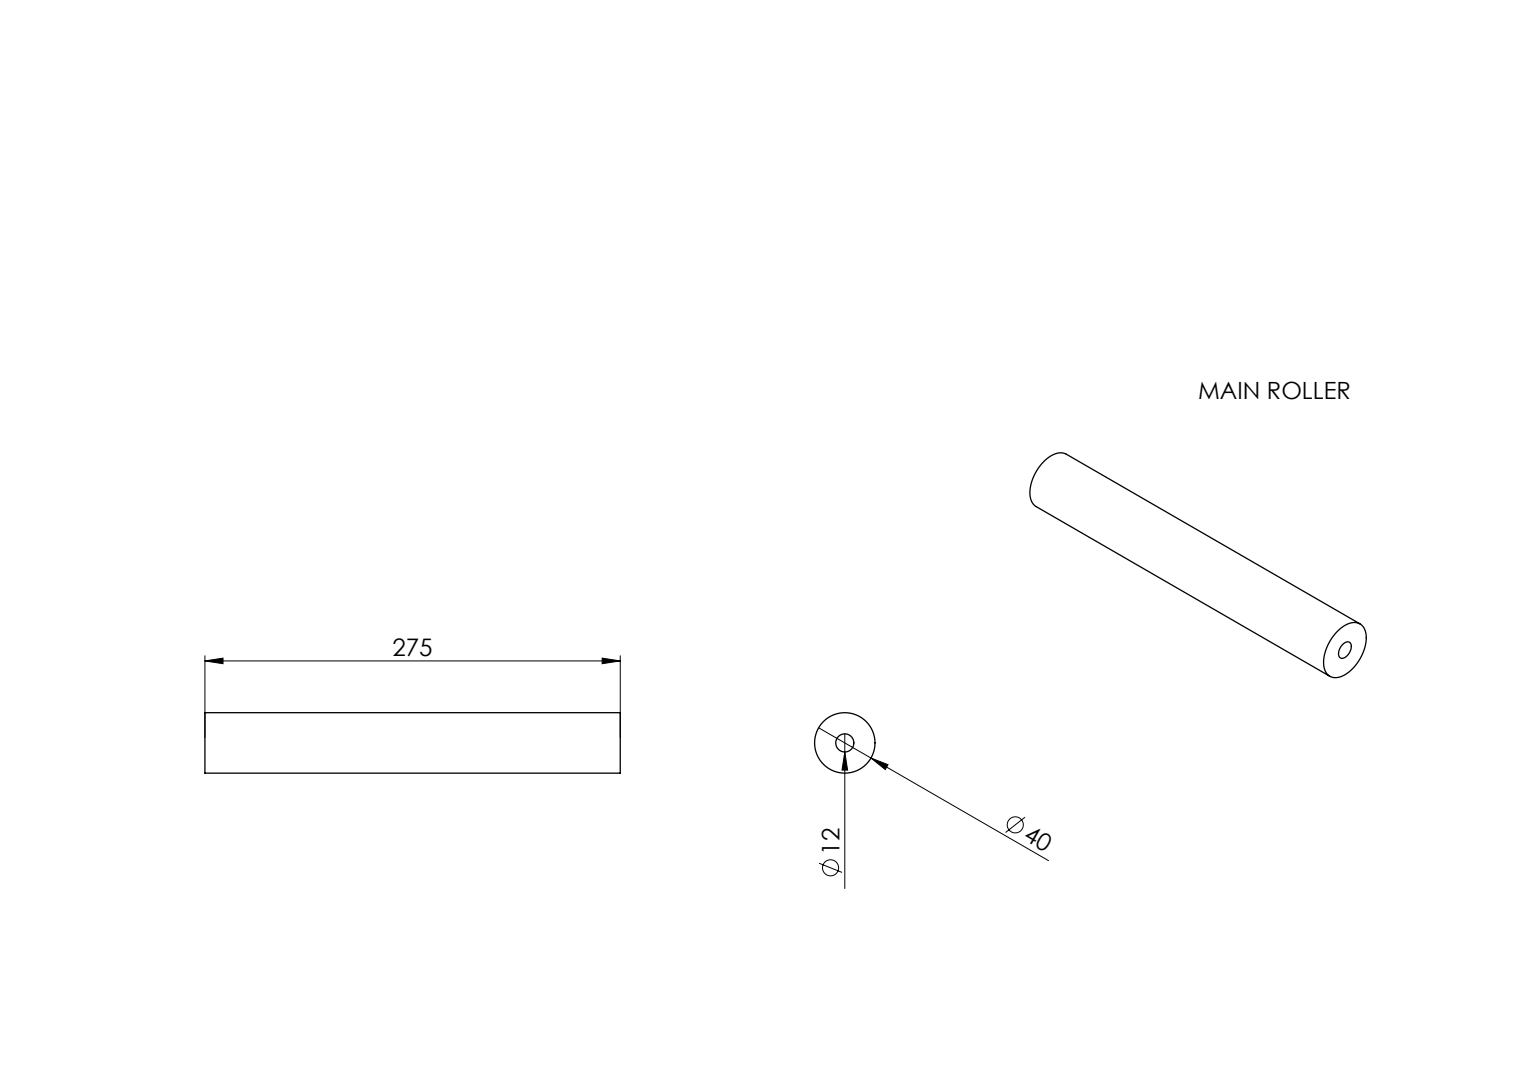
ISO-10303-21;
HEADER;
FILE_DESCRIPTION (('STEP AP214'),
    '1' );
FILE_NAME ('main roller.step',
    '2026-10-22T16:49:52',
    ( '' ),
    ( '' ),
    'SwSTEP 2.0',
    'SolidWorks 2026',
    '' );
FILE_SCHEMA (( 'AUTOMOTIVE_DESIGN' ));
ENDSEC;

DATA;
#49=CIRCLE ( 'NONE', #3968, 20.00000000000001421 ) ;
#63=CARTESIAN_POINT ( 'NONE',  ( 137.5000000000000000, 870.0000000000000000, 6.000000000000006217 ) ) ;
#76=CIRCLE ( 'NONE', #4758, 20.00000000000001421 ) ;
#77=AXIS2_PLACEMENT_3D ( 'NONE', #4332, #3953, #3470 ) ;
#109=APPLICATION_CONTEXT ( 'automotive_design' ) ;
#143=DIRECTION ( 'NONE',  ( 0.000000000000000000, 0.000000000000000000, -1.000000000000000000 ) ) ;
#179=EDGE_CURVE ( 'NONE', #353, #1195, #2907, .T. ) ;
#227=( GEOMETRIC_REPRESENTATION_CONTEXT ( 3 ) GLOBAL_UNCERTAINTY_ASSIGNED_CONTEXT ( ( #1775 ) ) GLOBAL_UNIT_ASSIGNED_CONTEXT ( ( #3570, #5196, #2363 ) ) REPRESENTATION_CONTEXT ( 'NONE', 'WORKASPACE' ) );
#245=CIRCLE ( 'NONE', #77, 6.000000000000006217 ) ;
#255=PRODUCT_DEFINITION ( 'UNKNOWN', '', #483, #2329 ) ;
#273=VERTEX_POINT ( 'NONE', #4446 ) ;
#291=EDGE_LOOP ( 'NONE', ( #3664, #547 ) ) ;
#309=CARTESIAN_POINT ( 'NONE',  ( -137.5000000000000000, 870.0000000000000000, 0.000000000000000000 ) ) ;
#332=DIRECTION ( 'NONE',  ( 0.000000000000000000, 0.000000000000000000, -1.000000000000000000 ) ) ;
#353=VERTEX_POINT ( 'NONE', #1576 ) ;
#387=ADVANCED_BREP_SHAPE_REPRESENTATION ( '', ( #3628, #4154 ), #755 ) ;
#405=MECHANICAL_DESIGN_GEOMETRIC_PRESENTATION_REPRESENTATION('',(#1277),#227);
#417=ORIENTED_EDGE ( 'NONE', *, *, #3310, .F. ) ;
#435=EDGE_CURVE ( 'NONE', #3050, #273, #1180, .T. ) ;
#479=ORIENTED_EDGE ( 'NONE', *, *, #5292, .T. ) ;
#483=PRODUCT_DEFINITION_FORMATION_WITH_SPECIFIED_SOURCE ( 'ANY', '', #4971, .NOT_KNOWN. ) ;
#496=FACE_BOUND ( 'NONE', #2841, .T. ) ;
#538=DIRECTION ( 'NONE',  ( 1.000000000000000000, 0.000000000000000000, 0.000000000000000000 ) ) ;
#547=ORIENTED_EDGE ( 'NONE', *, *, #2794, .F. ) ;
#562=VECTOR ( 'NONE', #3463, 1000.000000000000000 ) ;
#580=CARTESIAN_POINT ( 'NONE',  ( 137.5000000000000000, 870.0000000000000000, 0.000000000000000000 ) ) ;
#755=( GEOMETRIC_REPRESENTATION_CONTEXT ( 3 ) GLOBAL_UNCERTAINTY_ASSIGNED_CONTEXT ( ( #5058 ) ) GLOBAL_UNIT_ASSIGNED_CONTEXT ( ( #2393, #3976, #4011 ) ) REPRESENTATION_CONTEXT ( 'NONE', 'WORKASPACE' ) );
#769=DIRECTION ( 'NONE',  ( 1.000000000000000000, 0.000000000000000000, 0.000000000000000000 ) ) ;
#779=ADVANCED_FACE ( 'NONE', ( #1231 ), #2935, .T. ) ;
#808=DIRECTION ( 'NONE',  ( 0.000000000000000000, 0.000000000000000000, -1.000000000000000000 ) ) ;
#809=CARTESIAN_POINT ( 'NONE',  ( 137.5000000000000000, 870.0000000000000000, 0.000000000000000000 ) ) ;
#874=CYLINDRICAL_SURFACE ( 'NONE', #4672, 6.000000000000006217 ) ;
#913=AXIS2_PLACEMENT_3D ( 'NONE', #2357, #2823, #808 ) ;
#935=FACE_BOUND ( 'NONE', #291, .T. ) ;
#993=ORIENTED_EDGE ( 'NONE', *, *, #3708, .T. ) ;
#1058=ORIENTED_EDGE ( 'NONE', *, *, #1878, .F. ) ;
#1080=DIRECTION ( 'NONE',  ( 0.000000000000000000, 0.000000000000000000, -1.000000000000000000 ) ) ;
#1090=DIRECTION ( 'NONE',  ( 1.000000000000000000, 0.000000000000000000, 0.000000000000000000 ) ) ;
#1111=ORIENTED_EDGE ( 'NONE', *, *, #2237, .T. ) ;
#1112=DIRECTION ( 'NONE',  ( 1.000000000000000000, 0.000000000000000000, 0.000000000000000000 ) ) ;
#1150=ORIENTED_EDGE ( 'NONE', *, *, #179, .F. ) ;
#1180=LINE ( 'NONE', #3703, #3599 ) ;
#1184=AXIS2_PLACEMENT_3D ( 'NONE', #4858, #2059, #4475 ) ;
#1195=VERTEX_POINT ( 'NONE', #1817 ) ;
#1198=AXIS2_PLACEMENT_3D ( 'NONE', #4846, #4128, #332 ) ;
#1231=FACE_OUTER_BOUND ( 'NONE', #3832, .T. ) ;
#1232=CARTESIAN_POINT ( 'NONE',  ( 137.5000000000000000, 870.0000000000000000, 0.000000000000000000 ) ) ;
#1267=ORIENTED_EDGE ( 'NONE', *, *, #2794, .T. ) ;
#1270=CIRCLE ( 'NONE', #1184, 6.000000000000006217 ) ;
#1277=STYLED_ITEM ( 'NONE', ( #4776 ), #387 ) ;
#1282=FACE_OUTER_BOUND ( 'NONE', #2645, .T. ) ;
#1347=ADVANCED_FACE ( 'NONE', ( #3055, #496 ), #2097, .F. ) ;
#1502=AXIS2_PLACEMENT_3D ( 'NONE', #4105, #5347, #5379 ) ;
#1533=FILL_AREA_STYLE_COLOUR ( '', #4576 ) ;
#1549=SHAPE_DEFINITION_REPRESENTATION ( #4614, #3863 ) ;
#1568=CYLINDRICAL_SURFACE ( 'NONE', #2592, 20.00000000000001421 ) ;
#1576=CARTESIAN_POINT ( 'NONE',  ( 137.5000000000000000, 870.0000000000000000, -20.00000000000001421 ) ) ;
#1673=FACE_OUTER_BOUND ( 'NONE', #3685, .T. ) ;
#1728=EDGE_LOOP ( 'NONE', ( #417, #3099 ) ) ;
#1775=UNCERTAINTY_MEASURE_WITH_UNIT (LENGTH_MEASURE( 1.000000000000000082E-05 ), #3570, 'distance_accuracy_value', 'NONE');
#1778=LINE ( 'NONE', #5084, #562 ) ;
#1817=CARTESIAN_POINT ( 'NONE',  ( 137.5000000000000000, 870.0000000000000000, 20.00000000000001421 ) ) ;
#1876=( GEOMETRIC_REPRESENTATION_CONTEXT ( 3 ) GLOBAL_UNCERTAINTY_ASSIGNED_CONTEXT ( ( #4935 ) ) GLOBAL_UNIT_ASSIGNED_CONTEXT ( ( #4853, #2021, #4941 ) ) REPRESENTATION_CONTEXT ( 'NONE', 'WORKASPACE' ) );
#1878=EDGE_CURVE ( 'NONE', #1195, #353, #49, .T. ) ;
#1930=ORIENTED_EDGE ( 'NONE', *, *, #5007, .T. ) ;
#1934=DIRECTION ( 'NONE',  ( -1.000000000000000000, -0.000000000000000000, -0.000000000000000000 ) ) ;
#1974=FILL_AREA_STYLE ('',( #1533 ) ) ;
#2016=DIRECTION ( 'NONE',  ( 0.000000000000000000, 0.000000000000000000, -1.000000000000000000 ) ) ;
#2021=( NAMED_UNIT ( * ) PLANE_ANGLE_UNIT ( ) SI_UNIT ( $, .RADIAN. ) );
#2059=DIRECTION ( 'NONE',  ( 1.000000000000000000, 0.000000000000000000, 0.000000000000000000 ) ) ;
#2090=ORIENTED_EDGE ( 'NONE', *, *, #2811, .F. ) ;
#2097=PLANE ( 'NONE',  #4906 ) ;
#2145=VECTOR ( 'NONE', #3400, 1000.000000000000000 ) ;
#2150=DIRECTION ( 'NONE',  ( -1.000000000000000000, -0.000000000000000000, -0.000000000000000000 ) ) ;
#2237=EDGE_CURVE ( 'NONE', #1195, #4535, #1778, .T. ) ;
#2273=LINE ( 'NONE', #2360, #2755 ) ;
#2305=EDGE_CURVE ( 'NONE', #353, #4898, #2273, .T. ) ;
#2313=CIRCLE ( 'NONE', #913, 6.000000000000006217 ) ;
#2329=PRODUCT_DEFINITION_CONTEXT ( 'detailed design', #2921, 'design' ) ;
#2335=SURFACE_SIDE_STYLE ('',( #5281 ) ) ;
#2357=CARTESIAN_POINT ( 'NONE',  ( 137.5000000000000000, 870.0000000000000000, 0.000000000000000000 ) ) ;
#2360=CARTESIAN_POINT ( 'NONE',  ( 137.5000000000000000, 870.0000000000000000, -20.00000000000001421 ) ) ;
#2363=( NAMED_UNIT ( * ) SI_UNIT ( $, .STERADIAN. ) SOLID_ANGLE_UNIT ( ) );
#2393=( LENGTH_UNIT ( ) NAMED_UNIT ( * ) SI_UNIT ( .MILLI., .METRE. ) );
#2428=SHAPE_REPRESENTATION_RELATIONSHIP ( 'NONE' , 'NONE' ,  #3863, #387 ) ;
#2434=CARTESIAN_POINT ( 'NONE',  ( 0.000000000000000000, 0.000000000000000000, 0.000000000000000000 ) ) ;
#2473=EDGE_CURVE ( 'NONE', #3402, #273, #1270, .T. ) ;
#2545=CARTESIAN_POINT ( 'NONE',  ( 137.5000000000000000, 870.0000000000000000, 0.000000000000000000 ) ) ;
#2551=LINE ( 'NONE', #63, #2145 ) ;
#2553=CARTESIAN_POINT ( 'NONE',  ( 137.5000000000000000, 870.0000000000000000, -6.000000000000006217 ) ) ;
#2572=CARTESIAN_POINT ( 'NONE',  ( -137.5000000000000000, 870.0000000000000000, 0.000000000000000000 ) ) ;
#2592=AXIS2_PLACEMENT_3D ( 'NONE', #1232, #5380, #4932 ) ;
#2645=EDGE_LOOP ( 'NONE', ( #3636, #1267, #993, #2090 ) ) ;
#2665=CLOSED_SHELL ( 'NONE', ( #4635, #779, #4379, #1347, #3910, #5165 ) ) ;
#2684=ORIENTED_EDGE ( 'NONE', *, *, #1878, .T. ) ;
#2755=VECTOR ( 'NONE', #5251, 1000.000000000000000 ) ;
#2783=ORIENTED_EDGE ( 'NONE', *, *, #2305, .T. ) ;
#2794=EDGE_CURVE ( 'NONE', #3050, #4571, #2313, .T. ) ;
#2802=ORIENTED_EDGE ( 'NONE', *, *, #2473, .F. ) ;
#2811=EDGE_CURVE ( 'NONE', #273, #3402, #3638, .T. ) ;
#2823=DIRECTION ( 'NONE',  ( 1.000000000000000000, 0.000000000000000000, 0.000000000000000000 ) ) ;
#2841=EDGE_LOOP ( 'NONE', ( #4565, #4978 ) ) ;
#2887=PRODUCT_CONTEXT ( 'NONE', #109, 'mechanical' ) ;
#2907=CIRCLE ( 'NONE', #4273, 20.00000000000001421 ) ;
#2921=APPLICATION_CONTEXT ( 'automotive_design' ) ;
#2935=CYLINDRICAL_SURFACE ( 'NONE', #1502, 20.00000000000001421 ) ;
#2993=EDGE_LOOP ( 'NONE', ( #479, #5282, #2802, #4598 ) ) ;
#3017=DIRECTION ( 'NONE',  ( 0.000000000000000000, 0.000000000000000000, -1.000000000000000000 ) ) ;
#3045=DIRECTION ( 'NONE',  ( 1.000000000000000000, 0.000000000000000000, 0.000000000000000000 ) ) ;
#3050=VERTEX_POINT ( 'NONE', #2553 ) ;
#3055=FACE_OUTER_BOUND ( 'NONE', #1728, .T. ) ;
#3099=ORIENTED_EDGE ( 'NONE', *, *, #5007, .F. ) ;
#3107=CIRCLE ( 'NONE', #1198, 20.00000000000001421 ) ;
#3310=EDGE_CURVE ( 'NONE', #4535, #4898, #3107, .T. ) ;
#3351=ORIENTED_EDGE ( 'NONE', *, *, #3310, .T. ) ;
#3398=DIRECTION ( 'NONE',  ( 0.000000000000000000, 0.000000000000000000, -1.000000000000000000 ) ) ;
#3400=DIRECTION ( 'NONE',  ( -1.000000000000000000, -0.000000000000000000, -0.000000000000000000 ) ) ;
#3402=VERTEX_POINT ( 'NONE', #4961 ) ;
#3463=DIRECTION ( 'NONE',  ( -1.000000000000000000, -0.000000000000000000, -0.000000000000000000 ) ) ;
#3470=DIRECTION ( 'NONE',  ( 0.000000000000000000, 0.000000000000000000, -1.000000000000000000 ) ) ;
#3471=AXIS2_PLACEMENT_3D ( 'NONE', #809, #1934, #4911 ) ;
#3570=( LENGTH_UNIT ( ) NAMED_UNIT ( * ) SI_UNIT ( .MILLI., .METRE. ) );
#3599=VECTOR ( 'NONE', #5354, 1000.000000000000000 ) ;
#3628=MANIFOLD_SOLID_BREP ( 'Boss-Extrude1', #2665 ) ;
#3636=ORIENTED_EDGE ( 'NONE', *, *, #435, .F. ) ;
#3638=CIRCLE ( 'NONE', #5373, 6.000000000000006217 ) ;
#3655=DIRECTION ( 'NONE',  ( 1.000000000000000000, 0.000000000000000000, 0.000000000000000000 ) ) ;
#3664=ORIENTED_EDGE ( 'NONE', *, *, #5292, .F. ) ;
#3685=EDGE_LOOP ( 'NONE', ( #2684, #4617 ) ) ;
#3703=CARTESIAN_POINT ( 'NONE',  ( 137.5000000000000000, 870.0000000000000000, -6.000000000000006217 ) ) ;
#3705=CYLINDRICAL_SURFACE ( 'NONE', #3471, 6.000000000000006217 ) ;
#3708=EDGE_CURVE ( 'NONE', #4571, #3402, #2551, .T. ) ;
#3818=AXIS2_PLACEMENT_3D ( 'NONE', #5111, #3045, #3017 ) ;
#3825=DIRECTION ( 'NONE',  ( 0.000000000000000000, 0.000000000000000000, 1.000000000000000000 ) ) ;
#3832=EDGE_LOOP ( 'NONE', ( #1150, #2783, #1930, #5107 ) ) ;
#3836=PLANE ( 'NONE',  #3818 ) ;
#3863=SHAPE_REPRESENTATION ( 'main roller', ( #4154 ), #755 ) ;
#3885=DIRECTION ( 'NONE',  ( 1.000000000000000000, 0.000000000000000000, 0.000000000000000000 ) ) ;
#3910=ADVANCED_FACE ( 'NONE', ( #5324 ), #1568, .T. ) ;
#3933=CARTESIAN_POINT ( 'NONE',  ( -137.5000000000000000, 870.0000000000000000, -20.00000000000001421 ) ) ;
#3953=DIRECTION ( 'NONE',  ( 1.000000000000000000, 0.000000000000000000, 0.000000000000000000 ) ) ;
#3968=AXIS2_PLACEMENT_3D ( 'NONE', #4803, #1112, #1080 ) ;
#3976=( NAMED_UNIT ( * ) PLANE_ANGLE_UNIT ( ) SI_UNIT ( $, .RADIAN. ) );
#4011=( NAMED_UNIT ( * ) SI_UNIT ( $, .STERADIAN. ) SOLID_ANGLE_UNIT ( ) );
#4105=CARTESIAN_POINT ( 'NONE',  ( 137.5000000000000000, 870.0000000000000000, 0.000000000000000000 ) ) ;
#4114=FACE_OUTER_BOUND ( 'NONE', #2993, .T. ) ;
#4128=DIRECTION ( 'NONE',  ( 1.000000000000000000, 0.000000000000000000, 0.000000000000000000 ) ) ;
#4154=AXIS2_PLACEMENT_3D ( 'NONE', #2434, #5290, #769 ) ;
#4192=EDGE_LOOP ( 'NONE', ( #4956, #1058, #1111, #3351 ) ) ;
#4243=MECHANICAL_DESIGN_GEOMETRIC_PRESENTATION_REPRESENTATION('',(#5023),#1876);
#4273=AXIS2_PLACEMENT_3D ( 'NONE', #580, #3885, #143 ) ;
#4332=CARTESIAN_POINT ( 'NONE',  ( 137.5000000000000000, 870.0000000000000000, 0.000000000000000000 ) ) ;
#4369=CARTESIAN_POINT ( 'NONE',  ( -137.5000000000000000, 870.0000000000000000, 20.00000000000001421 ) ) ;
#4379=ADVANCED_FACE ( 'NONE', ( #1673, #935 ), #3836, .T. ) ;
#4446=CARTESIAN_POINT ( 'NONE',  ( -137.5000000000000000, 870.0000000000000000, -6.000000000000006217 ) ) ;
#4475=DIRECTION ( 'NONE',  ( 0.000000000000000000, 0.000000000000000000, -1.000000000000000000 ) ) ;
#4535=VERTEX_POINT ( 'NONE', #4369 ) ;
#4565=ORIENTED_EDGE ( 'NONE', *, *, #2473, .T. ) ;
#4571=VERTEX_POINT ( 'NONE', #5161 ) ;
#4576=COLOUR_RGB ( '',0.8941176470588234615, 0.8941176470588234615, 0.8941176470588234615 ) ;
#4598=ORIENTED_EDGE ( 'NONE', *, *, #3708, .F. ) ;
#4614=PRODUCT_DEFINITION_SHAPE ( 'NONE', 'NONE',  #255 ) ;
#4617=ORIENTED_EDGE ( 'NONE', *, *, #179, .T. ) ;
#4635=ADVANCED_FACE ( 'NONE', ( #4114 ), #3705, .F. ) ;
#4672=AXIS2_PLACEMENT_3D ( 'NONE', #2545, #2150, #3825 ) ;
#4758=AXIS2_PLACEMENT_3D ( 'NONE', #4875, #1090, #2016 ) ;
#4776=PRESENTATION_STYLE_ASSIGNMENT (( #5223 ) ) ;
#4803=CARTESIAN_POINT ( 'NONE',  ( 137.5000000000000000, 870.0000000000000000, 0.000000000000000000 ) ) ;
#4846=CARTESIAN_POINT ( 'NONE',  ( -137.5000000000000000, 870.0000000000000000, 0.000000000000000000 ) ) ;
#4853=( LENGTH_UNIT ( ) NAMED_UNIT ( * ) SI_UNIT ( .MILLI., .METRE. ) );
#4854=DIRECTION ( 'NONE',  ( 0.000000000000000000, 0.000000000000000000, -1.000000000000000000 ) ) ;
#4858=CARTESIAN_POINT ( 'NONE',  ( -137.5000000000000000, 870.0000000000000000, 0.000000000000000000 ) ) ;
#4875=CARTESIAN_POINT ( 'NONE',  ( -137.5000000000000000, 870.0000000000000000, 0.000000000000000000 ) ) ;
#4898=VERTEX_POINT ( 'NONE', #3933 ) ;
#4906=AXIS2_PLACEMENT_3D ( 'NONE', #2572, #538, #3398 ) ;
#4911=DIRECTION ( 'NONE',  ( 0.000000000000000000, 0.000000000000000000, 1.000000000000000000 ) ) ;
#4932=DIRECTION ( 'NONE',  ( 0.000000000000000000, 0.000000000000000000, 1.000000000000000000 ) ) ;
#4935=UNCERTAINTY_MEASURE_WITH_UNIT (LENGTH_MEASURE( 1.000000000000000082E-05 ), #4853, 'distance_accuracy_value', 'NONE');
#4941=( NAMED_UNIT ( * ) SI_UNIT ( $, .STERADIAN. ) SOLID_ANGLE_UNIT ( ) );
#4956=ORIENTED_EDGE ( 'NONE', *, *, #2305, .F. ) ;
#4961=CARTESIAN_POINT ( 'NONE',  ( -137.5000000000000000, 870.0000000000000000, 6.000000000000006217 ) ) ;
#4971=PRODUCT ( 'main roller', 'main roller', '', ( #2887 ) ) ;
#4978=ORIENTED_EDGE ( 'NONE', *, *, #2811, .T. ) ;
#5007=EDGE_CURVE ( 'NONE', #4898, #4535, #76, .T. ) ;
#5023=STYLED_ITEM('',(#5440),#3628);
#5058=UNCERTAINTY_MEASURE_WITH_UNIT (LENGTH_MEASURE( 1.000000000000000082E-05 ), #2393, 'distance_accuracy_value', 'NONE');
#5084=CARTESIAN_POINT ( 'NONE',  ( 137.5000000000000000, 870.0000000000000000, 20.00000000000001421 ) ) ;
#5107=ORIENTED_EDGE ( 'NONE', *, *, #2237, .F. ) ;
#5111=CARTESIAN_POINT ( 'NONE',  ( 137.5000000000000000, 870.0000000000000000, 0.000000000000000000 ) ) ;
#5161=CARTESIAN_POINT ( 'NONE',  ( 137.5000000000000000, 870.0000000000000000, 6.000000000000006217 ) ) ;
#5165=ADVANCED_FACE ( 'NONE', ( #1282 ), #874, .F. ) ;
#5196=( NAMED_UNIT ( * ) PLANE_ANGLE_UNIT ( ) SI_UNIT ( $, .RADIAN. ) );
#5223=SURFACE_STYLE_USAGE ( .BOTH. , #2335 ) ;
#5251=DIRECTION ( 'NONE',  ( -1.000000000000000000, -0.000000000000000000, -0.000000000000000000 ) ) ;
#5281=SURFACE_STYLE_FILL_AREA ( #1974 ) ;
#5282=ORIENTED_EDGE ( 'NONE', *, *, #435, .T. ) ;
#5290=DIRECTION ( 'NONE',  ( 0.000000000000000000, 0.000000000000000000, 1.000000000000000000 ) ) ;
#5292=EDGE_CURVE ( 'NONE', #4571, #3050, #245, .T. ) ;
#5324=FACE_OUTER_BOUND ( 'NONE', #4192, .T. ) ;
#5347=DIRECTION ( 'NONE',  ( -1.000000000000000000, -0.000000000000000000, -0.000000000000000000 ) ) ;
#5354=DIRECTION ( 'NONE',  ( -1.000000000000000000, -0.000000000000000000, -0.000000000000000000 ) ) ;
#5373=AXIS2_PLACEMENT_3D ( 'NONE', #309, #3655, #4854 ) ;
#5379=DIRECTION ( 'NONE',  ( 0.000000000000000000, 0.000000000000000000, 1.000000000000000000 ) ) ;
#5380=DIRECTION ( 'NONE',  ( -1.000000000000000000, -0.000000000000000000, -0.000000000000000000 ) ) ;
#5434=COLOUR_RGB('Off White',0.89,0.88,0.83);
#5435=FILL_AREA_STYLE_COLOUR('',#5434);
#5436=FILL_AREA_STYLE('',(#5435));
#5437=SURFACE_STYLE_FILL_AREA(#5436);
#5438=SURFACE_SIDE_STYLE('',(#5437));
#5439=SURFACE_STYLE_USAGE(.BOTH.,#5438);
#5440=PRESENTATION_STYLE_ASSIGNMENT((#5439));
ENDSEC;
END-ISO-10303-21;
